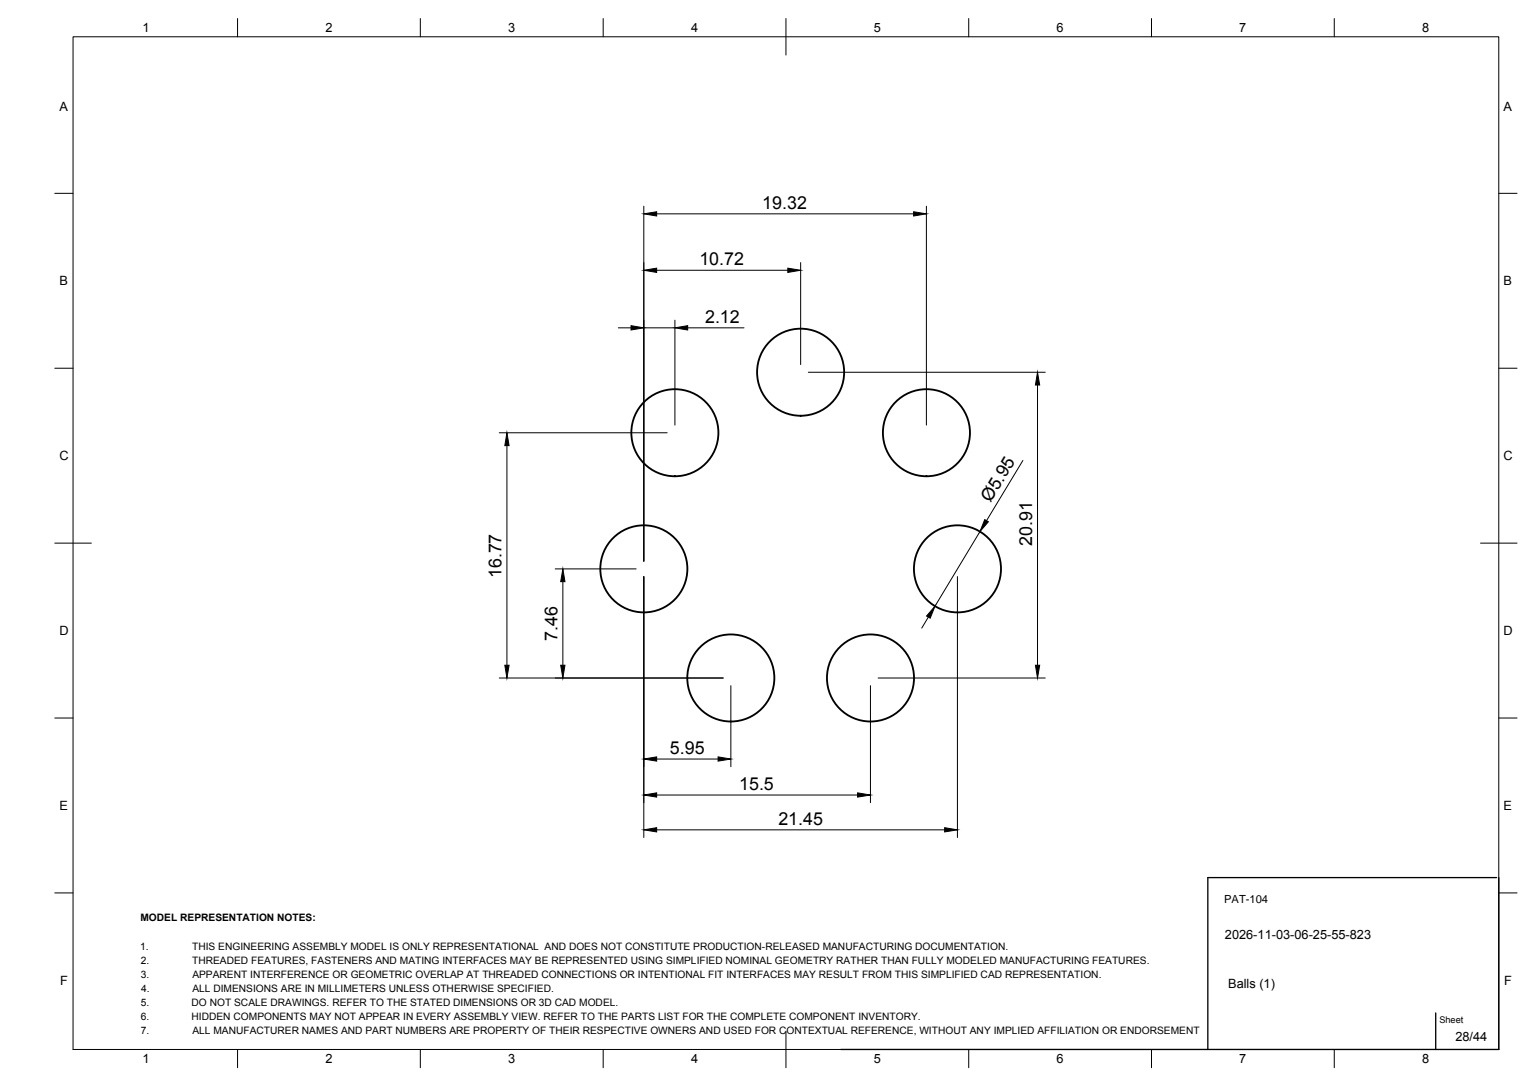
ISO-10303-21;
HEADER;
/* Generated by software containing ST-Developer
 * from STEP Tools, Inc. (www.steptools.com) 
 */

FILE_DESCRIPTION(
/* description */ ('Timing belt drive module 2 mm Pitch Timing 20T-40T'),

/* implementation_level */ '2;1');

FILE_NAME(
/* name */ 'Balls (1).step',
/* time_stamp */ '2026-10-28T03:25:12-07:00',
/* author */ (''),
/* organization */ (''),
/* preprocessor_version */ 'ST-DEVELOPER v20.2',
/* originating_system */ 'Autodesk Translation Framework v15.17.0.0',
/* authorisation */ '');

FILE_SCHEMA (('AUTOMOTIVE_DESIGN { 1 0 10303 214 3 1 1 }'));
ENDSEC;

DATA;
#10=MECHANICAL_DESIGN_GEOMETRIC_PRESENTATION_REPRESENTATION('',(#556,#557,#558,#559,#560,#561,#562),#17830);
#401=SPHERICAL_SURFACE('',#10082,0.29765);
#402=SPHERICAL_SURFACE('',#10084,0.29765);
#403=SPHERICAL_SURFACE('',#10086,0.29765);
#404=SPHERICAL_SURFACE('',#10088,0.29765);
#405=SPHERICAL_SURFACE('',#10090,0.29765);
#406=SPHERICAL_SURFACE('',#10092,0.29765);
#407=SPHERICAL_SURFACE('',#10094,0.29765);
#462=SHAPE_REPRESENTATION_RELATIONSHIP('SRR','None',#18034,#505);
#505=ADVANCED_BREP_SHAPE_REPRESENTATION('',(#613,#614,#615,#616,#617,#618,
#619),#17809);
#556=STYLED_ITEM('',(#18317),#613);
#557=STYLED_ITEM('',(#18317),#614);
#558=STYLED_ITEM('',(#18317),#615);
#559=STYLED_ITEM('',(#18317),#616);
#560=STYLED_ITEM('',(#18317),#617);
#561=STYLED_ITEM('',(#18317),#618);
#562=STYLED_ITEM('',(#18317),#619);
#613=MANIFOLD_SOLID_BREP('Body1',#9014);
#614=MANIFOLD_SOLID_BREP('Body2',#9015);
#615=MANIFOLD_SOLID_BREP('Body3',#9016);
#616=MANIFOLD_SOLID_BREP('Body4',#9017);
#617=MANIFOLD_SOLID_BREP('Body5',#9018);
#618=MANIFOLD_SOLID_BREP('Body6',#9019);
#619=MANIFOLD_SOLID_BREP('Body7',#9020);
#1214=FACE_OUTER_BOUND('',#1822,.T.);
#1215=FACE_OUTER_BOUND('',#1823,.T.);
#1216=FACE_OUTER_BOUND('',#1824,.T.);
#1217=FACE_OUTER_BOUND('',#1825,.T.);
#1218=FACE_OUTER_BOUND('',#1826,.T.);
#1219=FACE_OUTER_BOUND('',#1827,.T.);
#1220=FACE_OUTER_BOUND('',#1828,.T.);
#1822=EDGE_LOOP('',(#6887,#6888));
#1823=EDGE_LOOP('',(#6889,#6890));
#1824=EDGE_LOOP('',(#6891,#6892));
#1825=EDGE_LOOP('',(#6893,#6894));
#1826=EDGE_LOOP('',(#6895,#6896));
#1827=EDGE_LOOP('',(#6897,#6898));
#1828=EDGE_LOOP('',(#6899,#6900));
#2420=CIRCLE('',#10083,0.29765);
#2421=CIRCLE('',#10085,0.29765);
#2422=CIRCLE('',#10087,0.29765);
#2423=CIRCLE('',#10089,0.29765);
#2424=CIRCLE('',#10091,0.29765);
#2425=CIRCLE('',#10093,0.29765);
#2426=CIRCLE('',#10095,0.29765);
#4124=VERTEX_POINT('',#15433);
#4125=VERTEX_POINT('',#15434);
#4126=VERTEX_POINT('',#15437);
#4127=VERTEX_POINT('',#15438);
#4128=VERTEX_POINT('',#15441);
#4129=VERTEX_POINT('',#15442);
#4130=VERTEX_POINT('',#15445);
#4131=VERTEX_POINT('',#15446);
#4132=VERTEX_POINT('',#15449);
#4133=VERTEX_POINT('',#15450);
#4134=VERTEX_POINT('',#15453);
#4135=VERTEX_POINT('',#15454);
#4136=VERTEX_POINT('',#15457);
#4137=VERTEX_POINT('',#15458);
#5126=EDGE_CURVE('',#4124,#4125,#2420,.T.);
#5127=EDGE_CURVE('',#4126,#4127,#2421,.T.);
#5128=EDGE_CURVE('',#4128,#4129,#2422,.T.);
#5129=EDGE_CURVE('',#4130,#4131,#2423,.T.);
#5130=EDGE_CURVE('',#4132,#4133,#2424,.T.);
#5131=EDGE_CURVE('',#4134,#4135,#2425,.T.);
#5132=EDGE_CURVE('',#4136,#4137,#2426,.T.);
#6887=ORIENTED_EDGE('',*,*,#5126,.T.);
#6888=ORIENTED_EDGE('',*,*,#5126,.F.);
#6889=ORIENTED_EDGE('',*,*,#5127,.T.);
#6890=ORIENTED_EDGE('',*,*,#5127,.F.);
#6891=ORIENTED_EDGE('',*,*,#5128,.T.);
#6892=ORIENTED_EDGE('',*,*,#5128,.F.);
#6893=ORIENTED_EDGE('',*,*,#5129,.T.);
#6894=ORIENTED_EDGE('',*,*,#5129,.F.);
#6895=ORIENTED_EDGE('',*,*,#5130,.T.);
#6896=ORIENTED_EDGE('',*,*,#5130,.F.);
#6897=ORIENTED_EDGE('',*,*,#5131,.T.);
#6898=ORIENTED_EDGE('',*,*,#5131,.F.);
#6899=ORIENTED_EDGE('',*,*,#5132,.T.);
#6900=ORIENTED_EDGE('',*,*,#5132,.F.);
#8712=ADVANCED_FACE('',(#1214),#401,.T.);
#8713=ADVANCED_FACE('',(#1215),#402,.T.);
#8714=ADVANCED_FACE('',(#1216),#403,.T.);
#8715=ADVANCED_FACE('',(#1217),#404,.T.);
#8716=ADVANCED_FACE('',(#1218),#405,.T.);
#8717=ADVANCED_FACE('',(#1219),#406,.T.);
#8718=ADVANCED_FACE('',(#1220),#407,.T.);
#9014=CLOSED_SHELL('',(#8712));
#9015=CLOSED_SHELL('',(#8713));
#9016=CLOSED_SHELL('',(#8714));
#9017=CLOSED_SHELL('',(#8715));
#9018=CLOSED_SHELL('',(#8716));
#9019=CLOSED_SHELL('',(#8717));
#9020=CLOSED_SHELL('',(#8718));
#10081=AXIS2_PLACEMENT_3D('',#15431,#12198,#12199);
#10082=AXIS2_PLACEMENT_3D('',#15432,#12200,#12201);
#10083=AXIS2_PLACEMENT_3D('',#15435,#12202,#12203);
#10084=AXIS2_PLACEMENT_3D('',#15436,#12204,#12205);
#10085=AXIS2_PLACEMENT_3D('',#15439,#12206,#12207);
#10086=AXIS2_PLACEMENT_3D('',#15440,#12208,#12209);
#10087=AXIS2_PLACEMENT_3D('',#15443,#12210,#12211);
#10088=AXIS2_PLACEMENT_3D('',#15444,#12212,#12213);
#10089=AXIS2_PLACEMENT_3D('',#15447,#12214,#12215);
#10090=AXIS2_PLACEMENT_3D('',#15448,#12216,#12217);
#10091=AXIS2_PLACEMENT_3D('',#15451,#12218,#12219);
#10092=AXIS2_PLACEMENT_3D('',#15452,#12220,#12221);
#10093=AXIS2_PLACEMENT_3D('',#15455,#12222,#12223);
#10094=AXIS2_PLACEMENT_3D('',#15456,#12224,#12225);
#10095=AXIS2_PLACEMENT_3D('',#15459,#12226,#12227);
#12198=DIRECTION('axis',(0.,0.,1.));
#12199=DIRECTION('refdir',(1.,0.,0.));
#12200=DIRECTION('center_axis',(0.,0.,1.));
#12201=DIRECTION('ref_axis',(1.,0.,0.));
#12202=DIRECTION('center_axis',(1.22464679914735E-16,-1.,0.));
#12203=DIRECTION('ref_axis',(-1.,-1.22464679914735E-16,0.));
#12204=DIRECTION('center_axis',(0.78183148246803,0.,0.623489801858733));
#12205=DIRECTION('ref_axis',(0.623489801858734,0.,-0.78183148246803));
#12206=DIRECTION('center_axis',(7.63554790147315E-17,-1.,-9.57467422477103E-17));
#12207=DIRECTION('ref_axis',(-0.623489801858734,-1.22464679914735E-16,0.78183148246803));
#12208=DIRECTION('center_axis',(0.974927912181824,0.,-0.222520933956314));
#12209=DIRECTION('ref_axis',(-0.222520933956314,0.,-0.974927912181824));
#12210=DIRECTION('center_axis',(-2.7250954951288E-17,-1.,-1.19394234705288E-16));
#12211=DIRECTION('ref_axis',(0.222520933956314,-1.22464679914735E-16,0.974927912181824));
#12212=DIRECTION('center_axis',(0.433883739117558,0.,-0.900968867902419));
#12213=DIRECTION('ref_axis',(-0.900968867902419,0.,-0.433883739117558));
#12214=DIRECTION('center_axis',(-1.10336864020811E-16,-1.,-5.31354332312403E-17));
#12215=DIRECTION('ref_axis',(0.900968867902419,-1.22464679914735E-16,0.433883739117558));
#12216=DIRECTION('center_axis',(-0.433883739117558,0.,-0.900968867902419));
#12217=DIRECTION('ref_axis',(-0.900968867902419,0.,0.433883739117558));
#12218=DIRECTION('center_axis',(-1.10336864020811E-16,-1.,5.31354332312403E-17));
#12219=DIRECTION('ref_axis',(0.900968867902419,-1.22464679914735E-16,-0.433883739117558));
#12220=DIRECTION('center_axis',(-0.974927912181824,0.,-0.222520933956314));
#12221=DIRECTION('ref_axis',(-0.222520933956315,0.,0.974927912181824));
#12222=DIRECTION('center_axis',(-2.7250954951288E-17,-1.,1.19394234705288E-16));
#12223=DIRECTION('ref_axis',(0.222520933956315,-1.22464679914735E-16,-0.974927912181824));
#12224=DIRECTION('center_axis',(-0.78183148246803,0.,0.623489801858734));
#12225=DIRECTION('ref_axis',(0.623489801858733,0.,0.78183148246803));
#12226=DIRECTION('center_axis',(7.63554790147315E-17,-1.,9.57467422477103E-17));
#12227=DIRECTION('ref_axis',(-0.623489801858733,-1.22464679914735E-16,-0.78183148246803));
#15431=CARTESIAN_POINT('',(0.,0.,0.));
#15432=CARTESIAN_POINT('Origin',(1.1,0.,0.));
#15433=CARTESIAN_POINT('',(1.1,-2.23201749654651E-33,0.29765));
#15434=CARTESIAN_POINT('',(1.1,-2.23201749654651E-33,-0.29765));
#15435=CARTESIAN_POINT('Origin',(1.1,0.,0.));
#15436=CARTESIAN_POINT('Origin',(0.685838782044607,0.,-0.860014630714833));
#15437=CARTESIAN_POINT('',(0.918550922801216,-5.31350540756609E-33,-0.674432891191581));
#15438=CARTESIAN_POINT('',(0.453126641287998,8.49470414473068E-34,-1.04559637023808));
#15439=CARTESIAN_POINT('Origin',(0.685838782044607,0.,-0.860014630714833));
#15440=CARTESIAN_POINT('Origin',(-0.244773027351946,0.,-1.07242070340001));
#15441=CARTESIAN_POINT('',(0.0454142657089739,-2.23201749654651E-33,-1.1386540593921));
#15442=CARTESIAN_POINT('',(-0.534960320412865,-2.23201749654651E-33,-1.00618734740791));
#15443=CARTESIAN_POINT('Origin',(-0.244773027351946,0.,-1.07242070340001));
#15444=CARTESIAN_POINT('Origin',(-0.991065754692661,0.,-0.477272113029314));
#15445=CARTESIAN_POINT('',(-0.86192025974432,8.49470414473067E-34,-0.745445496560469));
#15446=CARTESIAN_POINT('',(-1.120211249641,-5.31350540756609E-33,-0.209098729498159));
#15447=CARTESIAN_POINT('Origin',(-0.991065754692661,0.,-0.477272113029314));
#15448=CARTESIAN_POINT('Origin',(-0.991065754692661,0.,0.477272113029314));
#15449=CARTESIAN_POINT('',(-1.120211249641,-2.23201749654651E-33,0.209098729498159));
#15450=CARTESIAN_POINT('',(-0.86192025974432,-2.23201749654651E-33,0.745445496560469));
#15451=CARTESIAN_POINT('Origin',(-0.991065754692661,0.,0.477272113029314));
#15452=CARTESIAN_POINT('Origin',(-0.244773027351946,0.,1.07242070340001));
#15453=CARTESIAN_POINT('',(-0.534960320412866,-2.23201749654651E-33,1.00618734740791));
#15454=CARTESIAN_POINT('',(0.0454142657089737,-2.23201749654651E-33,1.1386540593921));
#15455=CARTESIAN_POINT('Origin',(-0.244773027351946,0.,1.07242070340001));
#15456=CARTESIAN_POINT('Origin',(0.685838782044607,0.,0.860014630714833));
#15457=CARTESIAN_POINT('',(0.453126641287998,-2.23201749654651E-33,1.04559637023808));
#15458=CARTESIAN_POINT('',(0.918550922801216,-2.23201749654651E-33,0.674432891191581));
#15459=CARTESIAN_POINT('Origin',(0.685838782044607,0.,0.860014630714833));
#17759=UNCERTAINTY_MEASURE_WITH_UNIT(LENGTH_MEASURE(0.001),#17831,
'DISTANCE_ACCURACY_VALUE',
'Maximum model space distance between geometric entities at asserted c
onnectivities');
#17780=UNCERTAINTY_MEASURE_WITH_UNIT(LENGTH_MEASURE(0.001),#17831,
'DISTANCE_ACCURACY_VALUE',
'Maximum model space distance between geometric entities at asserted c
onnectivities');
#17809=(
GEOMETRIC_REPRESENTATION_CONTEXT(3)
GLOBAL_UNCERTAINTY_ASSIGNED_CONTEXT((#17759))
GLOBAL_UNIT_ASSIGNED_CONTEXT((#17831,#17833,#17834))
REPRESENTATION_CONTEXT('','3D')
);
#17830=(
GEOMETRIC_REPRESENTATION_CONTEXT(3)
GLOBAL_UNCERTAINTY_ASSIGNED_CONTEXT((#17780))
GLOBAL_UNIT_ASSIGNED_CONTEXT((#17831,#17833,#17834))
REPRESENTATION_CONTEXT('','3D')
);
#17831=(
LENGTH_UNIT()
NAMED_UNIT(*)
SI_UNIT(.CENTI.,.METRE.)
);
#17833=(
NAMED_UNIT(*)
PLANE_ANGLE_UNIT()
SI_UNIT($,.RADIAN.)
);
#17834=(
NAMED_UNIT(*)
SI_UNIT($,.STERADIAN.)
SOLID_ANGLE_UNIT()
);
#17863=SHAPE_DEFINITION_REPRESENTATION(#17917,#18034);
#17917=PRODUCT_DEFINITION_SHAPE('',$,#18084);
#18034=SHAPE_REPRESENTATION('',(#10081),#17809);
#18055=PRODUCT_DEFINITION_CONTEXT('part definition',#18204,'design');
#18084=PRODUCT_DEFINITION('Balls (1)','Balls (1)',#18133,#18055);
#18133=PRODUCT_DEFINITION_FORMATION('',$,#18234);
#18204=APPLICATION_CONTEXT(
'Core Data for Automotive Mechanical Design Process');
#18205=PRODUCT_CONTEXT('part definition',#18204,'mechanical');
#18234=PRODUCT('Balls (1)','Balls (1)','Balls (1)',(#18205));
#18311=COLOUR_RGB('Grey',0.48,0.52,0.57);
#18312=FILL_AREA_STYLE_COLOUR('',#18311);
#18313=FILL_AREA_STYLE('',(#18312));
#18314=SURFACE_STYLE_FILL_AREA(#18313);
#18315=SURFACE_SIDE_STYLE('',(#18314));
#18316=SURFACE_STYLE_USAGE(.BOTH.,#18315);
#18317=PRESENTATION_STYLE_ASSIGNMENT((#18316));
ENDSEC;
END-ISO-10303-21;
